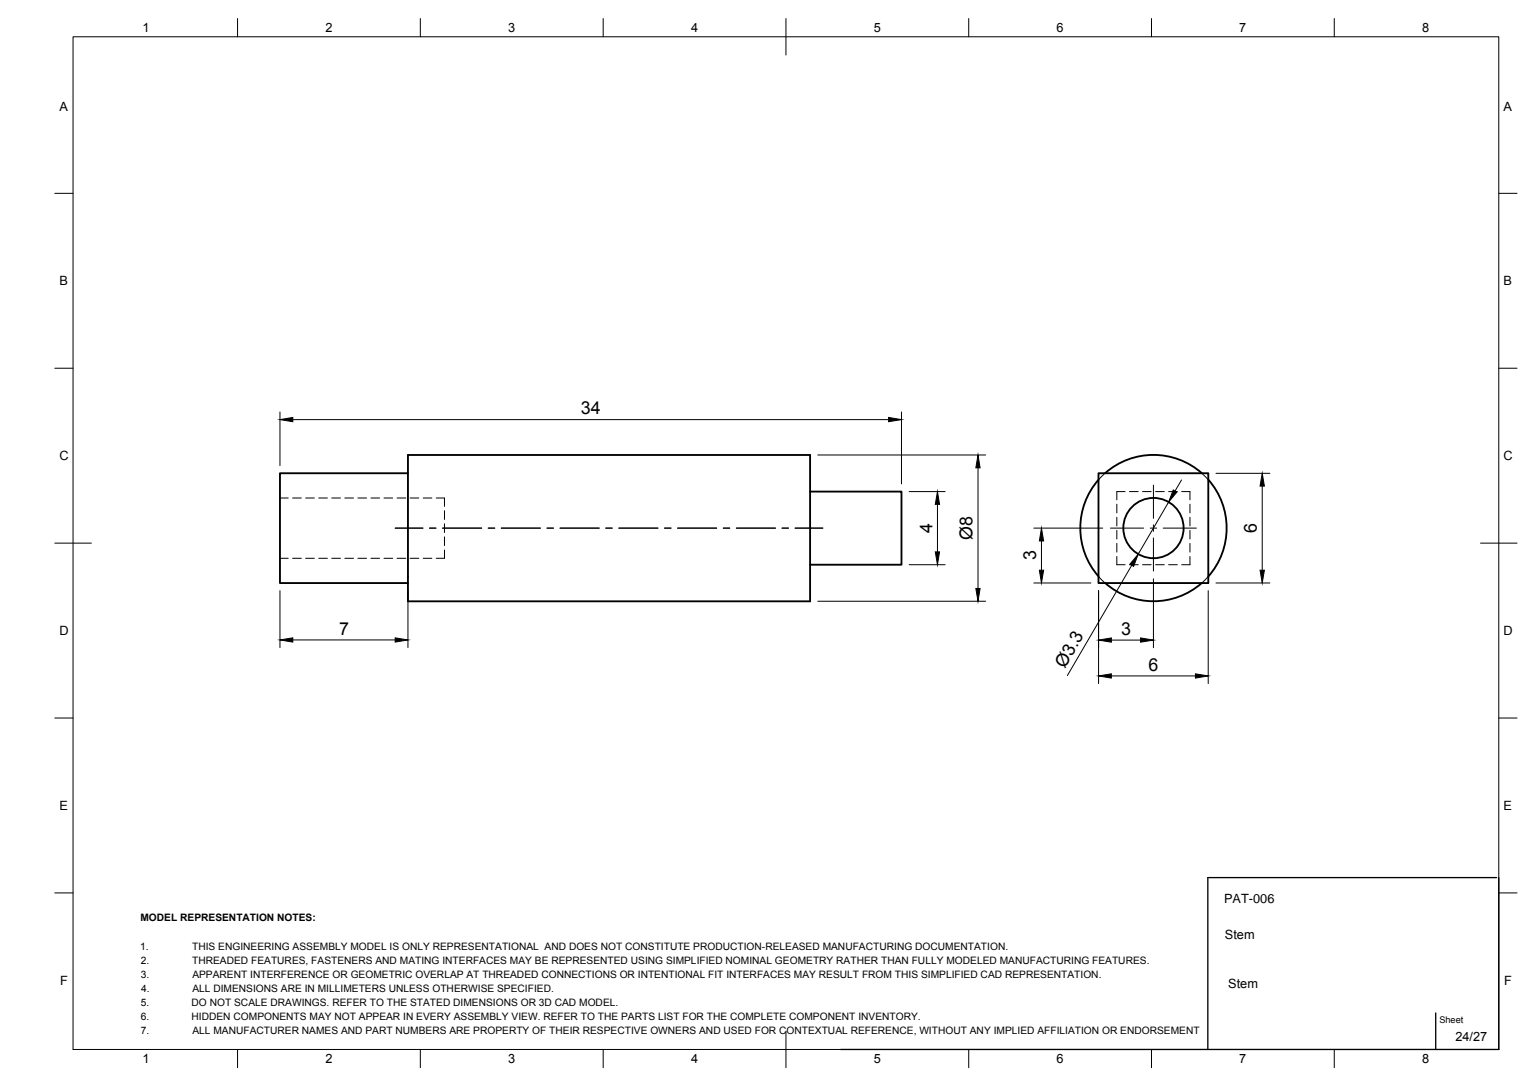
ISO-10303-21;
HEADER;
/* Generated by software containing ST-Developer
 * from STEP Tools, Inc. (www.steptools.com) 
 */

FILE_DESCRIPTION(
/* description */ ('Ball-type isolation valve (generic)'),
/* implementation_level */ '2;1');

FILE_NAME(
/* name */ 'Stem.step',
/* time_stamp */ '2026-10-27T10:53:05-07:00',
/* author */ (''),
/* organization */ (''),
/* preprocessor_version */ 'ST-DEVELOPER v20.2',
/* originating_system */ 'Autodesk Translation Framework v15.17.0.0',
/* authorisation */ '');

FILE_SCHEMA (('AUTOMOTIVE_DESIGN { 1 0 10303 214 3 1 1 }'));
ENDSEC;

DATA;
#10=MECHANICAL_DESIGN_GEOMETRIC_PRESENTATION_REPRESENTATION('',(#298),#7425);
#246=SHAPE_REPRESENTATION_RELATIONSHIP('SRR','None',#7557,#272);
#272=ADVANCED_BREP_SHAPE_REPRESENTATION('',(#322),#7420);
#298=STYLED_ITEM('',(#7737),#322);
#322=MANIFOLD_SOLID_BREP('Body1',#4105);
#412=FACE_BOUND('',#1111,.T.);
#413=FACE_BOUND('',#1123,.T.);
#530=PLANE('',#4806);
#531=PLANE('',#4807);
#532=PLANE('',#4809);
#533=PLANE('',#4811);
#534=PLANE('',#4813);
#535=PLANE('',#4815);
#536=PLANE('',#4816);
#537=PLANE('',#4817);
#538=PLANE('',#4818);
#539=PLANE('',#4819);
#540=PLANE('',#4820);
#541=PLANE('',#4822);
#542=PLANE('',#4825);
#543=PLANE('',#4827);
#544=PLANE('',#4829);
#545=PLANE('',#4830);
#546=PLANE('',#4831);
#547=PLANE('',#4832);
#548=PLANE('',#4833);
#549=PLANE('',#4836);
#770=FACE_OUTER_BOUND('',#1100,.T.);
#771=FACE_OUTER_BOUND('',#1101,.T.);
#772=FACE_OUTER_BOUND('',#1102,.T.);
#773=FACE_OUTER_BOUND('',#1103,.T.);
#774=FACE_OUTER_BOUND('',#1104,.T.);
#775=FACE_OUTER_BOUND('',#1105,.T.);
#776=FACE_OUTER_BOUND('',#1106,.T.);
#777=FACE_OUTER_BOUND('',#1107,.T.);
#778=FACE_OUTER_BOUND('',#1108,.T.);
#779=FACE_OUTER_BOUND('',#1109,.T.);
#780=FACE_OUTER_BOUND('',#1110,.T.);
#781=FACE_OUTER_BOUND('',#1112,.T.);
#782=FACE_OUTER_BOUND('',#1113,.T.);
#783=FACE_OUTER_BOUND('',#1114,.T.);
#784=FACE_OUTER_BOUND('',#1115,.T.);
#785=FACE_OUTER_BOUND('',#1116,.T.);
#786=FACE_OUTER_BOUND('',#1117,.T.);
#787=FACE_OUTER_BOUND('',#1118,.T.);
#788=FACE_OUTER_BOUND('',#1119,.T.);
#789=FACE_OUTER_BOUND('',#1120,.T.);
#790=FACE_OUTER_BOUND('',#1121,.T.);
#791=FACE_OUTER_BOUND('',#1122,.T.);
#1100=EDGE_LOOP('',(#3529,#3530,#3531,#3532));
#1101=EDGE_LOOP('',(#3533));
#1102=EDGE_LOOP('',(#3534,#3535,#3536));
#1103=EDGE_LOOP('',(#3537,#3538,#3539));
#1104=EDGE_LOOP('',(#3540,#3541,#3542));
#1105=EDGE_LOOP('',(#3543,#3544,#3545));
#1106=EDGE_LOOP('',(#3546,#3547,#3548,#3549,#3550,#3551));
#1107=EDGE_LOOP('',(#3552,#3553,#3554,#3555,#3556,#3557));
#1108=EDGE_LOOP('',(#3558,#3559,#3560,#3561,#3562,#3563));
#1109=EDGE_LOOP('',(#3564,#3565,#3566,#3567,#3568,#3569));
#1110=EDGE_LOOP('',(#3570,#3571,#3572,#3573));
#1111=EDGE_LOOP('',(#3574));
#1112=EDGE_LOOP('',(#3575,#3576));
#1113=EDGE_LOOP('',(#3577,#3578,#3579));
#1114=EDGE_LOOP('',(#3580,#3581));
#1115=EDGE_LOOP('',(#3582,#3583));
#1116=EDGE_LOOP('',(#3584,#3585,#3586,#3587));
#1117=EDGE_LOOP('',(#3588,#3589,#3590,#3591));
#1118=EDGE_LOOP('',(#3592,#3593,#3594,#3595));
#1119=EDGE_LOOP('',(#3596,#3597,#3598,#3599));
#1120=EDGE_LOOP('',(#3600,#3601,#3602,#3603));
#1121=EDGE_LOOP('',(#3604,#3605,#3606,#3607,#3608,#3609,#3610,#3611,#3612,
#3613,#3614,#3615));
#1122=EDGE_LOOP('',(#3616));
#1123=EDGE_LOOP('',(#3617,#3618,#3619,#3620));
#1378=LINE('',#7107,#1686);
#1379=LINE('',#7115,#1687);
#1380=LINE('',#7116,#1688);
#1381=LINE('',#7122,#1689);
#1382=LINE('',#7123,#1690);
#1383=LINE('',#7129,#1691);
#1384=LINE('',#7130,#1692);
#1385=LINE('',#7136,#1693);
#1386=LINE('',#7137,#1694);
#1387=LINE('',#7139,#1695);
#1388=LINE('',#7141,#1696);
#1389=LINE('',#7143,#1697);
#1390=LINE('',#7144,#1698);
#1391=LINE('',#7146,#1699);
#1392=LINE('',#7148,#1700);
#1393=LINE('',#7149,#1701);
#1394=LINE('',#7151,#1702);
#1395=LINE('',#7153,#1703);
#1396=LINE('',#7154,#1704);
#1397=LINE('',#7156,#1705);
#1398=LINE('',#7157,#1706);
#1399=LINE('',#7172,#1707);
#1400=LINE('',#7174,#1708);
#1401=LINE('',#7176,#1709);
#1402=LINE('',#7177,#1710);
#1403=LINE('',#7180,#1711);
#1404=LINE('',#7182,#1712);
#1405=LINE('',#7183,#1713);
#1406=LINE('',#7186,#1714);
#1407=LINE('',#7188,#1715);
#1408=LINE('',#7189,#1716);
#1409=LINE('',#7191,#1717);
#1410=LINE('',#7192,#1718);
#1411=LINE('',#7196,#1719);
#1686=VECTOR('',#5923,0.165);
#1687=VECTOR('',#5932,1.);
#1688=VECTOR('',#5933,1.);
#1689=VECTOR('',#5938,1.);
#1690=VECTOR('',#5939,1.);
#1691=VECTOR('',#5944,1.);
#1692=VECTOR('',#5945,1.);
#1693=VECTOR('',#5950,1.);
#1694=VECTOR('',#5951,1.);
#1695=VECTOR('',#5954,1.);
#1696=VECTOR('',#5955,1.);
#1697=VECTOR('',#5956,1.);
#1698=VECTOR('',#5957,1.);
#1699=VECTOR('',#5960,1.);
#1700=VECTOR('',#5961,1.);
#1701=VECTOR('',#5962,1.);
#1702=VECTOR('',#5965,1.);
#1703=VECTOR('',#5966,1.);
#1704=VECTOR('',#5967,1.);
#1705=VECTOR('',#5970,1.);
#1706=VECTOR('',#5971,1.);
#1707=VECTOR('',#5994,1.);
#1708=VECTOR('',#5995,1.);
#1709=VECTOR('',#5996,1.);
#1710=VECTOR('',#5997,1.);
#1711=VECTOR('',#6000,1.);
#1712=VECTOR('',#6001,1.);
#1713=VECTOR('',#6002,1.);
#1714=VECTOR('',#6005,1.);
#1715=VECTOR('',#6006,1.);
#1716=VECTOR('',#6007,1.);
#1717=VECTOR('',#6010,1.);
#1718=VECTOR('',#6011,1.);
#1719=VECTOR('',#6016,0.4);
#1933=CIRCLE('',#4804,0.165);
#1934=CIRCLE('',#4805,0.165);
#1935=CIRCLE('',#4808,0.4);
#1936=CIRCLE('',#4810,0.4);
#1937=CIRCLE('',#4812,0.4);
#1938=CIRCLE('',#4814,0.4);
#1939=CIRCLE('',#4821,0.4);
#1940=CIRCLE('',#4823,0.4);
#1941=CIRCLE('',#4824,0.4);
#1942=CIRCLE('',#4826,0.4);
#1943=CIRCLE('',#4828,0.4);
#1944=CIRCLE('',#4835,0.4);
#2205=VERTEX_POINT('',#7104);
#2206=VERTEX_POINT('',#7106);
#2207=VERTEX_POINT('',#7111);
#2208=VERTEX_POINT('',#7112);
#2209=VERTEX_POINT('',#7114);
#2210=VERTEX_POINT('',#7118);
#2211=VERTEX_POINT('',#7119);
#2212=VERTEX_POINT('',#7121);
#2213=VERTEX_POINT('',#7125);
#2214=VERTEX_POINT('',#7126);
#2215=VERTEX_POINT('',#7128);
#2216=VERTEX_POINT('',#7132);
#2217=VERTEX_POINT('',#7133);
#2218=VERTEX_POINT('',#7135);
#2219=VERTEX_POINT('',#7140);
#2220=VERTEX_POINT('',#7142);
#2221=VERTEX_POINT('',#7147);
#2222=VERTEX_POINT('',#7152);
#2223=VERTEX_POINT('',#7162);
#2224=VERTEX_POINT('',#7170);
#2225=VERTEX_POINT('',#7171);
#2226=VERTEX_POINT('',#7173);
#2227=VERTEX_POINT('',#7175);
#2228=VERTEX_POINT('',#7179);
#2229=VERTEX_POINT('',#7181);
#2230=VERTEX_POINT('',#7185);
#2231=VERTEX_POINT('',#7187);
#2232=VERTEX_POINT('',#7195);
#2657=EDGE_CURVE('',#2205,#2205,#1933,.T.);
#2658=EDGE_CURVE('',#2205,#2206,#1378,.T.);
#2659=EDGE_CURVE('',#2206,#2206,#1934,.T.);
#2660=EDGE_CURVE('',#2207,#2208,#1935,.T.);
#2661=EDGE_CURVE('',#2209,#2208,#1379,.T.);
#2662=EDGE_CURVE('',#2207,#2209,#1380,.T.);
#2663=EDGE_CURVE('',#2210,#2211,#1936,.T.);
#2664=EDGE_CURVE('',#2212,#2211,#1381,.T.);
#2665=EDGE_CURVE('',#2210,#2212,#1382,.T.);
#2666=EDGE_CURVE('',#2213,#2214,#1937,.T.);
#2667=EDGE_CURVE('',#2215,#2214,#1383,.T.);
#2668=EDGE_CURVE('',#2213,#2215,#1384,.T.);
#2669=EDGE_CURVE('',#2216,#2217,#1938,.T.);
#2670=EDGE_CURVE('',#2218,#2217,#1385,.T.);
#2671=EDGE_CURVE('',#2216,#2218,#1386,.T.);
#2672=EDGE_CURVE('',#2207,#2217,#1387,.T.);
#2673=EDGE_CURVE('',#2209,#2219,#1388,.T.);
#2674=EDGE_CURVE('',#2220,#2219,#1389,.T.);
#2675=EDGE_CURVE('',#2218,#2220,#1390,.T.);
#2676=EDGE_CURVE('',#2216,#2214,#1391,.T.);
#2677=EDGE_CURVE('',#2221,#2220,#1392,.T.);
#2678=EDGE_CURVE('',#2215,#2221,#1393,.T.);
#2679=EDGE_CURVE('',#2213,#2211,#1394,.T.);
#2680=EDGE_CURVE('',#2222,#2221,#1395,.T.);
#2681=EDGE_CURVE('',#2212,#2222,#1396,.T.);
#2682=EDGE_CURVE('',#2210,#2208,#1397,.T.);
#2683=EDGE_CURVE('',#2219,#2222,#1398,.T.);
#2684=EDGE_CURVE('',#2211,#2213,#1939,.T.);
#2685=EDGE_CURVE('',#2208,#2223,#1940,.T.);
#2686=EDGE_CURVE('',#2223,#2210,#1941,.T.);
#2687=EDGE_CURVE('',#2217,#2207,#1942,.T.);
#2688=EDGE_CURVE('',#2214,#2216,#1943,.T.);
#2689=EDGE_CURVE('',#2224,#2225,#1399,.T.);
#2690=EDGE_CURVE('',#2225,#2226,#1400,.T.);
#2691=EDGE_CURVE('',#2227,#2226,#1401,.T.);
#2692=EDGE_CURVE('',#2224,#2227,#1402,.T.);
#2693=EDGE_CURVE('',#2228,#2224,#1403,.T.);
#2694=EDGE_CURVE('',#2229,#2227,#1404,.T.);
#2695=EDGE_CURVE('',#2228,#2229,#1405,.T.);
#2696=EDGE_CURVE('',#2230,#2228,#1406,.T.);
#2697=EDGE_CURVE('',#2231,#2229,#1407,.T.);
#2698=EDGE_CURVE('',#2230,#2231,#1408,.T.);
#2699=EDGE_CURVE('',#2225,#2230,#1409,.T.);
#2700=EDGE_CURVE('',#2226,#2231,#1410,.T.);
#2701=EDGE_CURVE('',#2223,#2232,#1411,.T.);
#2702=EDGE_CURVE('',#2232,#2232,#1944,.T.);
#3529=ORIENTED_EDGE('',*,*,#2657,.F.);
#3530=ORIENTED_EDGE('',*,*,#2658,.T.);
#3531=ORIENTED_EDGE('',*,*,#2659,.F.);
#3532=ORIENTED_EDGE('',*,*,#2658,.F.);
#3533=ORIENTED_EDGE('',*,*,#2657,.T.);
#3534=ORIENTED_EDGE('',*,*,#2660,.T.);
#3535=ORIENTED_EDGE('',*,*,#2661,.F.);
#3536=ORIENTED_EDGE('',*,*,#2662,.F.);
#3537=ORIENTED_EDGE('',*,*,#2663,.T.);
#3538=ORIENTED_EDGE('',*,*,#2664,.F.);
#3539=ORIENTED_EDGE('',*,*,#2665,.F.);
#3540=ORIENTED_EDGE('',*,*,#2666,.T.);
#3541=ORIENTED_EDGE('',*,*,#2667,.F.);
#3542=ORIENTED_EDGE('',*,*,#2668,.F.);
#3543=ORIENTED_EDGE('',*,*,#2669,.T.);
#3544=ORIENTED_EDGE('',*,*,#2670,.F.);
#3545=ORIENTED_EDGE('',*,*,#2671,.F.);
#3546=ORIENTED_EDGE('',*,*,#2670,.T.);
#3547=ORIENTED_EDGE('',*,*,#2672,.F.);
#3548=ORIENTED_EDGE('',*,*,#2662,.T.);
#3549=ORIENTED_EDGE('',*,*,#2673,.T.);
#3550=ORIENTED_EDGE('',*,*,#2674,.F.);
#3551=ORIENTED_EDGE('',*,*,#2675,.F.);
#3552=ORIENTED_EDGE('',*,*,#2667,.T.);
#3553=ORIENTED_EDGE('',*,*,#2676,.F.);
#3554=ORIENTED_EDGE('',*,*,#2671,.T.);
#3555=ORIENTED_EDGE('',*,*,#2675,.T.);
#3556=ORIENTED_EDGE('',*,*,#2677,.F.);
#3557=ORIENTED_EDGE('',*,*,#2678,.F.);
#3558=ORIENTED_EDGE('',*,*,#2664,.T.);
#3559=ORIENTED_EDGE('',*,*,#2679,.F.);
#3560=ORIENTED_EDGE('',*,*,#2668,.T.);
#3561=ORIENTED_EDGE('',*,*,#2678,.T.);
#3562=ORIENTED_EDGE('',*,*,#2680,.F.);
#3563=ORIENTED_EDGE('',*,*,#2681,.F.);
#3564=ORIENTED_EDGE('',*,*,#2661,.T.);
#3565=ORIENTED_EDGE('',*,*,#2682,.F.);
#3566=ORIENTED_EDGE('',*,*,#2665,.T.);
#3567=ORIENTED_EDGE('',*,*,#2681,.T.);
#3568=ORIENTED_EDGE('',*,*,#2683,.F.);
#3569=ORIENTED_EDGE('',*,*,#2673,.F.);
#3570=ORIENTED_EDGE('',*,*,#2683,.T.);
#3571=ORIENTED_EDGE('',*,*,#2680,.T.);
#3572=ORIENTED_EDGE('',*,*,#2677,.T.);
#3573=ORIENTED_EDGE('',*,*,#2674,.T.);
#3574=ORIENTED_EDGE('',*,*,#2659,.T.);
#3575=ORIENTED_EDGE('',*,*,#2679,.T.);
#3576=ORIENTED_EDGE('',*,*,#2684,.T.);
#3577=ORIENTED_EDGE('',*,*,#2682,.T.);
#3578=ORIENTED_EDGE('',*,*,#2685,.T.);
#3579=ORIENTED_EDGE('',*,*,#2686,.T.);
#3580=ORIENTED_EDGE('',*,*,#2672,.T.);
#3581=ORIENTED_EDGE('',*,*,#2687,.T.);
#3582=ORIENTED_EDGE('',*,*,#2676,.T.);
#3583=ORIENTED_EDGE('',*,*,#2688,.T.);
#3584=ORIENTED_EDGE('',*,*,#2689,.T.);
#3585=ORIENTED_EDGE('',*,*,#2690,.T.);
#3586=ORIENTED_EDGE('',*,*,#2691,.F.);
#3587=ORIENTED_EDGE('',*,*,#2692,.F.);
#3588=ORIENTED_EDGE('',*,*,#2693,.T.);
#3589=ORIENTED_EDGE('',*,*,#2692,.T.);
#3590=ORIENTED_EDGE('',*,*,#2694,.F.);
#3591=ORIENTED_EDGE('',*,*,#2695,.F.);
#3592=ORIENTED_EDGE('',*,*,#2696,.T.);
#3593=ORIENTED_EDGE('',*,*,#2695,.T.);
#3594=ORIENTED_EDGE('',*,*,#2697,.F.);
#3595=ORIENTED_EDGE('',*,*,#2698,.F.);
#3596=ORIENTED_EDGE('',*,*,#2699,.T.);
#3597=ORIENTED_EDGE('',*,*,#2698,.T.);
#3598=ORIENTED_EDGE('',*,*,#2700,.F.);
#3599=ORIENTED_EDGE('',*,*,#2690,.F.);
#3600=ORIENTED_EDGE('',*,*,#2699,.F.);
#3601=ORIENTED_EDGE('',*,*,#2689,.F.);
#3602=ORIENTED_EDGE('',*,*,#2693,.F.);
#3603=ORIENTED_EDGE('',*,*,#2696,.F.);
#3604=ORIENTED_EDGE('',*,*,#2685,.F.);
#3605=ORIENTED_EDGE('',*,*,#2660,.F.);
#3606=ORIENTED_EDGE('',*,*,#2687,.F.);
#3607=ORIENTED_EDGE('',*,*,#2669,.F.);
#3608=ORIENTED_EDGE('',*,*,#2688,.F.);
#3609=ORIENTED_EDGE('',*,*,#2666,.F.);
#3610=ORIENTED_EDGE('',*,*,#2684,.F.);
#3611=ORIENTED_EDGE('',*,*,#2663,.F.);
#3612=ORIENTED_EDGE('',*,*,#2686,.F.);
#3613=ORIENTED_EDGE('',*,*,#2701,.T.);
#3614=ORIENTED_EDGE('',*,*,#2702,.T.);
#3615=ORIENTED_EDGE('',*,*,#2701,.F.);
#3616=ORIENTED_EDGE('',*,*,#2702,.F.);
#3617=ORIENTED_EDGE('',*,*,#2691,.T.);
#3618=ORIENTED_EDGE('',*,*,#2700,.T.);
#3619=ORIENTED_EDGE('',*,*,#2697,.T.);
#3620=ORIENTED_EDGE('',*,*,#2694,.T.);
#3827=CYLINDRICAL_SURFACE('',#4803,0.165);
#3828=CYLINDRICAL_SURFACE('',#4834,0.4);
#4024=ADVANCED_FACE('',(#770),#3827,.F.);
#4025=ADVANCED_FACE('',(#771),#530,.T.);
#4026=ADVANCED_FACE('',(#772),#531,.F.);
#4027=ADVANCED_FACE('',(#773),#532,.F.);
#4028=ADVANCED_FACE('',(#774),#533,.F.);
#4029=ADVANCED_FACE('',(#775),#534,.F.);
#4030=ADVANCED_FACE('',(#776),#535,.T.);
#4031=ADVANCED_FACE('',(#777),#536,.T.);
#4032=ADVANCED_FACE('',(#778),#537,.T.);
#4033=ADVANCED_FACE('',(#779),#538,.T.);
#4034=ADVANCED_FACE('',(#780,#412),#539,.T.);
#4035=ADVANCED_FACE('',(#781),#540,.T.);
#4036=ADVANCED_FACE('',(#782),#541,.T.);
#4037=ADVANCED_FACE('',(#783),#542,.T.);
#4038=ADVANCED_FACE('',(#784),#543,.T.);
#4039=ADVANCED_FACE('',(#785),#544,.T.);
#4040=ADVANCED_FACE('',(#786),#545,.T.);
#4041=ADVANCED_FACE('',(#787),#546,.T.);
#4042=ADVANCED_FACE('',(#788),#547,.T.);
#4043=ADVANCED_FACE('',(#789),#548,.F.);
#4044=ADVANCED_FACE('',(#790),#3828,.T.);
#4045=ADVANCED_FACE('',(#791,#413),#549,.F.);
#4105=CLOSED_SHELL('',(#4024,#4025,#4026,#4027,#4028,#4029,#4030,#4031,
#4032,#4033,#4034,#4035,#4036,#4037,#4038,#4039,#4040,#4041,#4042,#4043,
#4044,#4045));
#4802=AXIS2_PLACEMENT_3D('',#7102,#5917,#5918);
#4803=AXIS2_PLACEMENT_3D('',#7103,#5919,#5920);
#4804=AXIS2_PLACEMENT_3D('',#7105,#5921,#5922);
#4805=AXIS2_PLACEMENT_3D('',#7108,#5924,#5925);
#4806=AXIS2_PLACEMENT_3D('',#7109,#5926,#5927);
#4807=AXIS2_PLACEMENT_3D('',#7110,#5928,#5929);
#4808=AXIS2_PLACEMENT_3D('',#7113,#5930,#5931);
#4809=AXIS2_PLACEMENT_3D('',#7117,#5934,#5935);
#4810=AXIS2_PLACEMENT_3D('',#7120,#5936,#5937);
#4811=AXIS2_PLACEMENT_3D('',#7124,#5940,#5941);
#4812=AXIS2_PLACEMENT_3D('',#7127,#5942,#5943);
#4813=AXIS2_PLACEMENT_3D('',#7131,#5946,#5947);
#4814=AXIS2_PLACEMENT_3D('',#7134,#5948,#5949);
#4815=AXIS2_PLACEMENT_3D('',#7138,#5952,#5953);
#4816=AXIS2_PLACEMENT_3D('',#7145,#5958,#5959);
#4817=AXIS2_PLACEMENT_3D('',#7150,#5963,#5964);
#4818=AXIS2_PLACEMENT_3D('',#7155,#5968,#5969);
#4819=AXIS2_PLACEMENT_3D('',#7158,#5972,#5973);
#4820=AXIS2_PLACEMENT_3D('',#7159,#5974,#5975);
#4821=AXIS2_PLACEMENT_3D('',#7160,#5976,#5977);
#4822=AXIS2_PLACEMENT_3D('',#7161,#5978,#5979);
#4823=AXIS2_PLACEMENT_3D('',#7163,#5980,#5981);
#4824=AXIS2_PLACEMENT_3D('',#7164,#5982,#5983);
#4825=AXIS2_PLACEMENT_3D('',#7165,#5984,#5985);
#4826=AXIS2_PLACEMENT_3D('',#7166,#5986,#5987);
#4827=AXIS2_PLACEMENT_3D('',#7167,#5988,#5989);
#4828=AXIS2_PLACEMENT_3D('',#7168,#5990,#5991);
#4829=AXIS2_PLACEMENT_3D('',#7169,#5992,#5993);
#4830=AXIS2_PLACEMENT_3D('',#7178,#5998,#5999);
#4831=AXIS2_PLACEMENT_3D('',#7184,#6003,#6004);
#4832=AXIS2_PLACEMENT_3D('',#7190,#6008,#6009);
#4833=AXIS2_PLACEMENT_3D('',#7193,#6012,#6013);
#4834=AXIS2_PLACEMENT_3D('',#7194,#6014,#6015);
#4835=AXIS2_PLACEMENT_3D('',#7197,#6017,#6018);
#4836=AXIS2_PLACEMENT_3D('',#7198,#6019,#6020);
#5917=DIRECTION('axis',(0.,0.,1.));
#5918=DIRECTION('refdir',(1.,0.,0.));
#5919=DIRECTION('center_axis',(0.,0.,1.));
#5920=DIRECTION('ref_axis',(1.,0.,0.));
#5921=DIRECTION('center_axis',(0.,0.,1.));
#5922=DIRECTION('ref_axis',(1.,0.,0.));
#5923=DIRECTION('',(0.,0.,1.));
#5924=DIRECTION('center_axis',(0.,0.,-1.));
#5925=DIRECTION('ref_axis',(1.,0.,0.));
#5926=DIRECTION('center_axis',(0.,0.,1.));
#5927=DIRECTION('ref_axis',(1.,0.,0.));
#5928=DIRECTION('center_axis',(0.,0.,1.));
#5929=DIRECTION('ref_axis',(1.,0.,0.));
#5930=DIRECTION('center_axis',(0.,0.,1.));
#5931=DIRECTION('ref_axis',(1.,0.,0.));
#5932=DIRECTION('',(0.,-1.,0.));
#5933=DIRECTION('',(-1.,0.,0.));
#5934=DIRECTION('center_axis',(0.,0.,1.));
#5935=DIRECTION('ref_axis',(1.,0.,0.));
#5936=DIRECTION('center_axis',(0.,0.,1.));
#5937=DIRECTION('ref_axis',(1.,0.,0.));
#5938=DIRECTION('',(1.,0.,0.));
#5939=DIRECTION('',(0.,-1.,0.));
#5940=DIRECTION('center_axis',(0.,0.,1.));
#5941=DIRECTION('ref_axis',(1.,0.,0.));
#5942=DIRECTION('center_axis',(0.,0.,1.));
#5943=DIRECTION('ref_axis',(1.,0.,0.));
#5944=DIRECTION('',(0.,1.,0.));
#5945=DIRECTION('',(1.,0.,0.));
#5946=DIRECTION('center_axis',(0.,0.,1.));
#5947=DIRECTION('ref_axis',(1.,0.,0.));
#5948=DIRECTION('center_axis',(0.,0.,1.));
#5949=DIRECTION('ref_axis',(1.,0.,0.));
#5950=DIRECTION('',(-1.,0.,0.));
#5951=DIRECTION('',(0.,1.,0.));
#5952=DIRECTION('center_axis',(0.,1.,0.));
#5953=DIRECTION('ref_axis',(-1.,0.,0.));
#5954=DIRECTION('',(1.,0.,0.));
#5955=DIRECTION('',(0.,0.,1.));
#5956=DIRECTION('',(-1.,0.,0.));
#5957=DIRECTION('',(0.,0.,1.));
#5958=DIRECTION('center_axis',(1.,0.,0.));
#5959=DIRECTION('ref_axis',(0.,1.,0.));
#5960=DIRECTION('',(0.,-1.,0.));
#5961=DIRECTION('',(0.,1.,0.));
#5962=DIRECTION('',(0.,0.,1.));
#5963=DIRECTION('center_axis',(0.,-1.,0.));
#5964=DIRECTION('ref_axis',(1.,0.,0.));
#5965=DIRECTION('',(-1.,0.,0.));
#5966=DIRECTION('',(1.,0.,0.));
#5967=DIRECTION('',(0.,0.,1.));
#5968=DIRECTION('center_axis',(-1.,0.,0.));
#5969=DIRECTION('ref_axis',(0.,-1.,0.));
#5970=DIRECTION('',(0.,1.,0.));
#5971=DIRECTION('',(0.,-1.,0.));
#5972=DIRECTION('center_axis',(0.,0.,1.));
#5973=DIRECTION('ref_axis',(1.,0.,0.));
#5974=DIRECTION('center_axis',(0.,0.,1.));
#5975=DIRECTION('ref_axis',(1.,0.,0.));
#5976=DIRECTION('center_axis',(0.,0.,1.));
#5977=DIRECTION('ref_axis',(1.,0.,0.));
#5978=DIRECTION('center_axis',(0.,0.,1.));
#5979=DIRECTION('ref_axis',(1.,0.,0.));
#5980=DIRECTION('center_axis',(0.,0.,1.));
#5981=DIRECTION('ref_axis',(1.,0.,0.));
#5982=DIRECTION('center_axis',(0.,0.,1.));
#5983=DIRECTION('ref_axis',(1.,0.,0.));
#5984=DIRECTION('center_axis',(0.,0.,1.));
#5985=DIRECTION('ref_axis',(1.,0.,0.));
#5986=DIRECTION('center_axis',(0.,0.,1.));
#5987=DIRECTION('ref_axis',(1.,0.,0.));
#5988=DIRECTION('center_axis',(0.,0.,1.));
#5989=DIRECTION('ref_axis',(1.,0.,0.));
#5990=DIRECTION('center_axis',(0.,0.,1.));
#5991=DIRECTION('ref_axis',(1.,0.,0.));
#5992=DIRECTION('center_axis',(0.,1.,0.));
#5993=DIRECTION('ref_axis',(-1.,0.,0.));
#5994=DIRECTION('',(-1.,0.,0.));
#5995=DIRECTION('',(0.,0.,1.));
#5996=DIRECTION('',(-1.,0.,0.));
#5997=DIRECTION('',(0.,0.,1.));
#5998=DIRECTION('center_axis',(1.,0.,0.));
#5999=DIRECTION('ref_axis',(0.,1.,0.));
#6000=DIRECTION('',(0.,1.,0.));
#6001=DIRECTION('',(0.,1.,0.));
#6002=DIRECTION('',(0.,0.,1.));
#6003=DIRECTION('center_axis',(0.,-1.,0.));
#6004=DIRECTION('ref_axis',(1.,0.,0.));
#6005=DIRECTION('',(1.,0.,0.));
#6006=DIRECTION('',(1.,0.,0.));
#6007=DIRECTION('',(0.,0.,1.));
#6008=DIRECTION('center_axis',(-1.,0.,0.));
#6009=DIRECTION('ref_axis',(0.,-1.,0.));
#6010=DIRECTION('',(0.,-1.,0.));
#6011=DIRECTION('',(0.,-1.,0.));
#6012=DIRECTION('center_axis',(0.,0.,1.));
#6013=DIRECTION('ref_axis',(1.,0.,0.));
#6014=DIRECTION('center_axis',(0.,0.,1.));
#6015=DIRECTION('ref_axis',(1.,0.,0.));
#6016=DIRECTION('',(0.,0.,-1.));
#6017=DIRECTION('center_axis',(0.,0.,1.));
#6018=DIRECTION('ref_axis',(1.,0.,0.));
#6019=DIRECTION('center_axis',(0.,0.,1.));
#6020=DIRECTION('ref_axis',(1.,0.,0.));
#7102=CARTESIAN_POINT('',(0.,0.,0.));
#7103=CARTESIAN_POINT('Origin',(0.,0.,8.5));
#7104=CARTESIAN_POINT('',(-0.165,-2.02066721859313E-17,8.5));
#7105=CARTESIAN_POINT('Origin',(0.,0.,8.5));
#7106=CARTESIAN_POINT('',(-0.165,2.02066721859313E-17,9.4));
#7107=CARTESIAN_POINT('',(-0.165,-2.02066721859313E-17,8.5));
#7108=CARTESIAN_POINT('Origin',(0.,0.,9.4));
#7109=CARTESIAN_POINT('Origin',(0.,0.,8.5));
#7110=CARTESIAN_POINT('Origin',(0.,0.,8.7));
#7111=CARTESIAN_POINT('',(-0.264575131106459,0.3,8.7));
#7112=CARTESIAN_POINT('',(-0.3,0.264575131106459,8.7));
#7113=CARTESIAN_POINT('Origin',(0.,0.,8.7));
#7114=CARTESIAN_POINT('',(-0.3,0.3,8.7));
#7115=CARTESIAN_POINT('',(-0.3,0.3,8.7));
#7116=CARTESIAN_POINT('',(0.3,0.3,8.7));
#7117=CARTESIAN_POINT('Origin',(0.,0.,8.7));
#7118=CARTESIAN_POINT('',(-0.3,-0.264575131106459,8.7));
#7119=CARTESIAN_POINT('',(-0.264575131106459,-0.3,8.7));
#7120=CARTESIAN_POINT('Origin',(0.,0.,8.7));
#7121=CARTESIAN_POINT('',(-0.3,-0.3,8.7));
#7122=CARTESIAN_POINT('',(-0.3,-0.3,8.7));
#7123=CARTESIAN_POINT('',(-0.3,0.3,8.7));
#7124=CARTESIAN_POINT('Origin',(0.,0.,8.7));
#7125=CARTESIAN_POINT('',(0.264575131106459,-0.3,8.7));
#7126=CARTESIAN_POINT('',(0.3,-0.264575131106459,8.7));
#7127=CARTESIAN_POINT('Origin',(0.,0.,8.7));
#7128=CARTESIAN_POINT('',(0.3,-0.3,8.7));
#7129=CARTESIAN_POINT('',(0.3,-0.3,8.7));
#7130=CARTESIAN_POINT('',(-0.3,-0.3,8.7));
#7131=CARTESIAN_POINT('Origin',(0.,0.,8.7));
#7132=CARTESIAN_POINT('',(0.3,0.264575131106459,8.7));
#7133=CARTESIAN_POINT('',(0.264575131106459,0.3,8.7));
#7134=CARTESIAN_POINT('Origin',(0.,0.,8.7));
#7135=CARTESIAN_POINT('',(0.3,0.3,8.7));
#7136=CARTESIAN_POINT('',(0.3,0.3,8.7));
#7137=CARTESIAN_POINT('',(0.3,-0.3,8.7));
#7138=CARTESIAN_POINT('Origin',(0.3,0.3,8.7));
#7139=CARTESIAN_POINT('',(0.15,0.3,8.7));
#7140=CARTESIAN_POINT('',(-0.3,0.3,9.4));
#7141=CARTESIAN_POINT('',(-0.3,0.3,8.7));
#7142=CARTESIAN_POINT('',(0.3,0.3,9.4));
#7143=CARTESIAN_POINT('',(0.3,0.3,9.4));
#7144=CARTESIAN_POINT('',(0.3,0.3,8.7));
#7145=CARTESIAN_POINT('Origin',(0.3,-0.3,8.7));
#7146=CARTESIAN_POINT('',(0.3,-0.15,8.7));
#7147=CARTESIAN_POINT('',(0.3,-0.3,9.4));
#7148=CARTESIAN_POINT('',(0.3,-0.3,9.4));
#7149=CARTESIAN_POINT('',(0.3,-0.3,8.7));
#7150=CARTESIAN_POINT('Origin',(-0.3,-0.3,8.7));
#7151=CARTESIAN_POINT('',(-0.15,-0.3,8.7));
#7152=CARTESIAN_POINT('',(-0.3,-0.3,9.4));
#7153=CARTESIAN_POINT('',(-0.3,-0.3,9.4));
#7154=CARTESIAN_POINT('',(-0.3,-0.3,8.7));
#7155=CARTESIAN_POINT('Origin',(-0.3,0.3,8.7));
#7156=CARTESIAN_POINT('',(-0.3,0.15,8.7));
#7157=CARTESIAN_POINT('',(-0.3,0.3,9.4));
#7158=CARTESIAN_POINT('Origin',(0.,0.,9.4));
#7159=CARTESIAN_POINT('Origin',(0.,0.,8.7));
#7160=CARTESIAN_POINT('Origin',(0.,0.,8.7));
#7161=CARTESIAN_POINT('Origin',(0.,0.,8.7));
#7162=CARTESIAN_POINT('',(-0.4,-4.89858719658941E-17,8.7));
#7163=CARTESIAN_POINT('Origin',(0.,0.,8.7));
#7164=CARTESIAN_POINT('Origin',(0.,0.,8.7));
#7165=CARTESIAN_POINT('Origin',(0.,0.,8.7));
#7166=CARTESIAN_POINT('Origin',(0.,0.,8.7));
#7167=CARTESIAN_POINT('Origin',(0.,0.,8.7));
#7168=CARTESIAN_POINT('Origin',(0.,0.,8.7));
#7169=CARTESIAN_POINT('Origin',(0.2,0.2,6.));
#7170=CARTESIAN_POINT('',(0.2,0.2,6.));
#7171=CARTESIAN_POINT('',(-0.2,0.2,6.));
#7172=CARTESIAN_POINT('',(0.2,0.2,6.));
#7173=CARTESIAN_POINT('',(-0.2,0.2,6.5));
#7174=CARTESIAN_POINT('',(-0.2,0.2,6.));
#7175=CARTESIAN_POINT('',(0.2,0.2,6.5));
#7176=CARTESIAN_POINT('',(0.1,0.2,6.5));
#7177=CARTESIAN_POINT('',(0.2,0.2,6.));
#7178=CARTESIAN_POINT('Origin',(0.2,-0.2,6.));
#7179=CARTESIAN_POINT('',(0.2,-0.2,6.));
#7180=CARTESIAN_POINT('',(0.2,-0.2,6.));
#7181=CARTESIAN_POINT('',(0.2,-0.2,6.5));
#7182=CARTESIAN_POINT('',(0.2,-0.1,6.5));
#7183=CARTESIAN_POINT('',(0.2,-0.2,6.));
#7184=CARTESIAN_POINT('Origin',(-0.2,-0.2,6.));
#7185=CARTESIAN_POINT('',(-0.2,-0.2,6.));
#7186=CARTESIAN_POINT('',(-0.2,-0.2,6.));
#7187=CARTESIAN_POINT('',(-0.2,-0.2,6.5));
#7188=CARTESIAN_POINT('',(-0.1,-0.2,6.5));
#7189=CARTESIAN_POINT('',(-0.2,-0.2,6.));
#7190=CARTESIAN_POINT('Origin',(-0.2,0.2,6.));
#7191=CARTESIAN_POINT('',(-0.2,0.2,6.));
#7192=CARTESIAN_POINT('',(-0.2,0.1,6.5));
#7193=CARTESIAN_POINT('Origin',(0.,0.,6.));
#7194=CARTESIAN_POINT('Origin',(0.,0.,6.5));
#7195=CARTESIAN_POINT('',(-0.4,-4.89858719658941E-17,6.5));
#7196=CARTESIAN_POINT('',(-0.4,-4.89858719658941E-17,6.5));
#7197=CARTESIAN_POINT('Origin',(0.,0.,6.5));
#7198=CARTESIAN_POINT('Origin',(0.,0.,6.5));
#7390=UNCERTAINTY_MEASURE_WITH_UNIT(LENGTH_MEASURE(0.001),#7426,
'DISTANCE_ACCURACY_VALUE',
'Maximum model space distance between geometric entities at asserted c
onnectivities');
#7395=UNCERTAINTY_MEASURE_WITH_UNIT(LENGTH_MEASURE(0.001),#7426,
'DISTANCE_ACCURACY_VALUE',
'Maximum model space distance between geometric entities at asserted c
onnectivities');
#7420=(
GEOMETRIC_REPRESENTATION_CONTEXT(3)
GLOBAL_UNCERTAINTY_ASSIGNED_CONTEXT((#7390))
GLOBAL_UNIT_ASSIGNED_CONTEXT((#7426,#7428,#7429))
REPRESENTATION_CONTEXT('','3D')
);
#7425=(
GEOMETRIC_REPRESENTATION_CONTEXT(3)
GLOBAL_UNCERTAINTY_ASSIGNED_CONTEXT((#7395))
GLOBAL_UNIT_ASSIGNED_CONTEXT((#7426,#7428,#7429))
REPRESENTATION_CONTEXT('','3D')
);
#7426=(
LENGTH_UNIT()
NAMED_UNIT(*)
SI_UNIT(.CENTI.,.METRE.)
);
#7428=(
NAMED_UNIT(*)
PLANE_ANGLE_UNIT()
SI_UNIT($,.RADIAN.)
);
#7429=(
NAMED_UNIT(*)
SI_UNIT($,.STERADIAN.)
SOLID_ANGLE_UNIT()
);
#7454=SHAPE_DEFINITION_REPRESENTATION(#7520,#7557);
#7520=PRODUCT_DEFINITION_SHAPE('',$,#7587);
#7557=SHAPE_REPRESENTATION('',(#4802),#7420);
#7562=PRODUCT_DEFINITION_CONTEXT('part definition',#7651,'design');
#7587=PRODUCT_DEFINITION('Stem','Stem',#7616,#7562);
#7616=PRODUCT_DEFINITION_FORMATION('',$,#7677);
#7651=APPLICATION_CONTEXT(
'Core Data for Automotive Mechanical Design Process');
#7652=PRODUCT_CONTEXT('part definition',#7651,'mechanical');
#7677=PRODUCT('Stem','Stem','Stem',(#7652));
#7731=COLOUR_RGB('Sky Blue',0.24,0.69,0.87);
#7732=FILL_AREA_STYLE_COLOUR('',#7731);
#7733=FILL_AREA_STYLE('',(#7732));
#7734=SURFACE_STYLE_FILL_AREA(#7733);
#7735=SURFACE_SIDE_STYLE('',(#7734));
#7736=SURFACE_STYLE_USAGE(.BOTH.,#7735);
#7737=PRESENTATION_STYLE_ASSIGNMENT((#7736));
ENDSEC;
END-ISO-10303-21;
